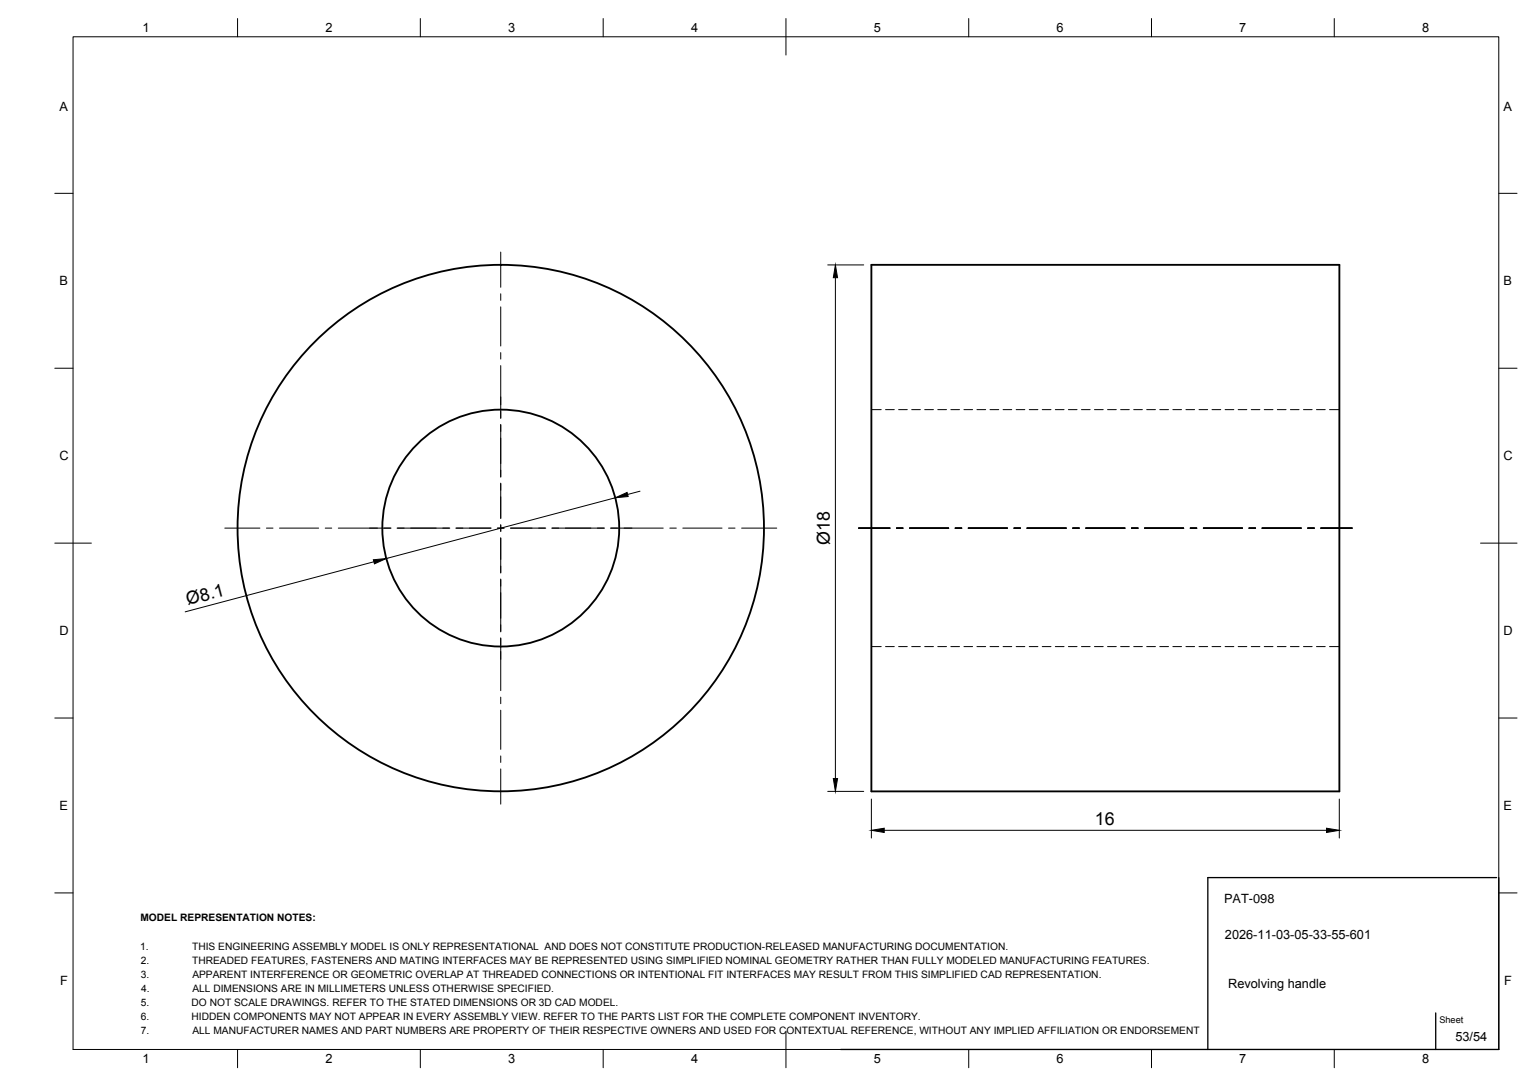
ISO-10303-21;
HEADER;
/* Generated by software containing ST-Developer
 * from STEP Tools, Inc. (www.steptools.com) 
 */

FILE_DESCRIPTION(
/* description */ ('Spring compression tester'),
/* implementation_level */ '2;1');

FILE_NAME(
/* name */ 'Revolving handle.step',
/* time_stamp */ '2026-10-28T03:24:11-07:00',
/* author */ (''),
/* organization */ (''),
/* preprocessor_version */ 'ST-DEVELOPER v20.2',
/* originating_system */ 'Autodesk Translation Framework v15.17.0.0',
/* authorisation */ '');

FILE_SCHEMA (('AUTOMOTIVE_DESIGN { 1 0 10303 214 3 1 1 }'));
ENDSEC;

DATA;
#10=MECHANICAL_DESIGN_GEOMETRIC_PRESENTATION_REPRESENTATION('',(#1174),#43521);
#1039=SHAPE_REPRESENTATION_RELATIONSHIP('SRR','None',#43856,#1099);
#1099=ADVANCED_BREP_SHAPE_REPRESENTATION('',(#1243),#43516);
#1174=STYLED_ITEM('',(#44195),#1243);
#1243=MANIFOLD_SOLID_BREP('Body1',#18617);
#1583=FACE_BOUND('',#4556,.T.);
#1584=FACE_BOUND('',#4558,.T.);
#2136=PLANE('',#21117);
#2137=PLANE('',#21118);
#3170=FACE_OUTER_BOUND('',#4553,.T.);
#3171=FACE_OUTER_BOUND('',#4554,.T.);
#3172=FACE_OUTER_BOUND('',#4555,.T.);
#3173=FACE_OUTER_BOUND('',#4557,.T.);
#4553=EDGE_LOOP('',(#16919,#16920,#16921,#16922));
#4554=EDGE_LOOP('',(#16923,#16924,#16925,#16926));
#4555=EDGE_LOOP('',(#16927));
#4556=EDGE_LOOP('',(#16928));
#4557=EDGE_LOOP('',(#16929));
#4558=EDGE_LOOP('',(#16930));
#5965=LINE('',#43172,#7397);
#5966=LINE('',#43178,#7398);
#7397=VECTOR('',#26213,0.405);
#7398=VECTOR('',#26220,0.9);
#8116=CIRCLE('',#21112,0.405);
#8117=CIRCLE('',#21113,0.405);
#8118=CIRCLE('',#21115,0.9);
#8119=CIRCLE('',#21116,0.9);
#9713=VERTEX_POINT('',#43169);
#9714=VERTEX_POINT('',#43171);
#9715=VERTEX_POINT('',#43175);
#9716=VERTEX_POINT('',#43177);
#12124=EDGE_CURVE('',#9713,#9713,#8116,.T.);
#12125=EDGE_CURVE('',#9713,#9714,#5965,.T.);
#12126=EDGE_CURVE('',#9714,#9714,#8117,.T.);
#12127=EDGE_CURVE('',#9715,#9715,#8118,.T.);
#12128=EDGE_CURVE('',#9715,#9716,#5966,.T.);
#12129=EDGE_CURVE('',#9716,#9716,#8119,.T.);
#16919=ORIENTED_EDGE('',*,*,#12124,.F.);
#16920=ORIENTED_EDGE('',*,*,#12125,.T.);
#16921=ORIENTED_EDGE('',*,*,#12126,.T.);
#16922=ORIENTED_EDGE('',*,*,#12125,.F.);
#16923=ORIENTED_EDGE('',*,*,#12127,.F.);
#16924=ORIENTED_EDGE('',*,*,#12128,.T.);
#16925=ORIENTED_EDGE('',*,*,#12129,.T.);
#16926=ORIENTED_EDGE('',*,*,#12128,.F.);
#16927=ORIENTED_EDGE('',*,*,#12127,.T.);
#16928=ORIENTED_EDGE('',*,*,#12124,.T.);
#16929=ORIENTED_EDGE('',*,*,#12129,.F.);
#16930=ORIENTED_EDGE('',*,*,#12126,.F.);
#17487=CYLINDRICAL_SURFACE('',#21111,0.405);
#17488=CYLINDRICAL_SURFACE('',#21114,0.9);
#18494=ADVANCED_FACE('',(#3170),#17487,.F.);
#18495=ADVANCED_FACE('',(#3171),#17488,.T.);
#18496=ADVANCED_FACE('',(#3172,#1583),#2136,.T.);
#18497=ADVANCED_FACE('',(#3173,#1584),#2137,.F.);
#18617=CLOSED_SHELL('',(#18494,#18495,#18496,#18497));
#21110=AXIS2_PLACEMENT_3D('',#43167,#26207,#26208);
#21111=AXIS2_PLACEMENT_3D('',#43168,#26209,#26210);
#21112=AXIS2_PLACEMENT_3D('',#43170,#26211,#26212);
#21113=AXIS2_PLACEMENT_3D('',#43173,#26214,#26215);
#21114=AXIS2_PLACEMENT_3D('',#43174,#26216,#26217);
#21115=AXIS2_PLACEMENT_3D('',#43176,#26218,#26219);
#21116=AXIS2_PLACEMENT_3D('',#43179,#26221,#26222);
#21117=AXIS2_PLACEMENT_3D('',#43180,#26223,#26224);
#21118=AXIS2_PLACEMENT_3D('',#43181,#26225,#26226);
#26207=DIRECTION('axis',(0.,0.,1.));
#26208=DIRECTION('refdir',(1.,0.,0.));
#26209=DIRECTION('center_axis',(1.,0.,0.));
#26210=DIRECTION('ref_axis',(0.,0.,-1.));
#26211=DIRECTION('center_axis',(-1.,0.,0.));
#26212=DIRECTION('ref_axis',(0.,0.,-1.));
#26213=DIRECTION('',(-1.,0.,0.));
#26214=DIRECTION('center_axis',(-1.,0.,0.));
#26215=DIRECTION('ref_axis',(0.,0.,-1.));
#26216=DIRECTION('center_axis',(1.,0.,0.));
#26217=DIRECTION('ref_axis',(0.,0.,-1.));
#26218=DIRECTION('center_axis',(1.,0.,0.));
#26219=DIRECTION('ref_axis',(0.,0.,-1.));
#26220=DIRECTION('',(-1.,0.,0.));
#26221=DIRECTION('center_axis',(1.,0.,0.));
#26222=DIRECTION('ref_axis',(0.,0.,-1.));
#26223=DIRECTION('center_axis',(1.,0.,0.));
#26224=DIRECTION('ref_axis',(0.,0.,-1.));
#26225=DIRECTION('center_axis',(1.,0.,0.));
#26226=DIRECTION('ref_axis',(0.,0.,-1.));
#43167=CARTESIAN_POINT('',(0.,0.,0.));
#43168=CARTESIAN_POINT('Origin',(29.4,0.,6.5));
#43169=CARTESIAN_POINT('',(31.,-4.95981953654678E-17,6.905));
#43170=CARTESIAN_POINT('Origin',(31.,0.,6.5));
#43171=CARTESIAN_POINT('',(29.4,-4.95981953654678E-17,6.905));
#43172=CARTESIAN_POINT('',(29.4,-4.95981953654678E-17,6.905));
#43173=CARTESIAN_POINT('Origin',(29.4,0.,6.5));
#43174=CARTESIAN_POINT('Origin',(29.4,0.,6.5));
#43175=CARTESIAN_POINT('',(31.,-1.10218211923262E-16,7.4));
#43176=CARTESIAN_POINT('Origin',(31.,0.,6.5));
#43177=CARTESIAN_POINT('',(29.4,-1.10218211923262E-16,7.4));
#43178=CARTESIAN_POINT('',(29.4,-1.10218211923262E-16,7.4));
#43179=CARTESIAN_POINT('Origin',(29.4,0.,6.5));
#43180=CARTESIAN_POINT('Origin',(31.,0.,6.5));
#43181=CARTESIAN_POINT('Origin',(29.4,0.,6.5));
#43448=UNCERTAINTY_MEASURE_WITH_UNIT(LENGTH_MEASURE(0.001),#43522,
'DISTANCE_ACCURACY_VALUE',
'Maximum model space distance between geometric entities at asserted c
onnectivities');
#43453=UNCERTAINTY_MEASURE_WITH_UNIT(LENGTH_MEASURE(0.001),#43522,
'DISTANCE_ACCURACY_VALUE',
'Maximum model space distance between geometric entities at asserted c
onnectivities');
#43516=(
GEOMETRIC_REPRESENTATION_CONTEXT(3)
GLOBAL_UNCERTAINTY_ASSIGNED_CONTEXT((#43448))
GLOBAL_UNIT_ASSIGNED_CONTEXT((#43522,#43524,#43525))
REPRESENTATION_CONTEXT('','3D')
);
#43521=(
GEOMETRIC_REPRESENTATION_CONTEXT(3)
GLOBAL_UNCERTAINTY_ASSIGNED_CONTEXT((#43453))
GLOBAL_UNIT_ASSIGNED_CONTEXT((#43522,#43524,#43525))
REPRESENTATION_CONTEXT('','3D')
);
#43522=(
LENGTH_UNIT()
NAMED_UNIT(*)
SI_UNIT(.CENTI.,.METRE.)
);
#43524=(
NAMED_UNIT(*)
PLANE_ANGLE_UNIT()
SI_UNIT($,.RADIAN.)
);
#43525=(
NAMED_UNIT(*)
SI_UNIT($,.STERADIAN.)
SOLID_ANGLE_UNIT()
);
#43588=SHAPE_DEFINITION_REPRESENTATION(#43775,#43856);
#43775=PRODUCT_DEFINITION_SHAPE('',$,#43924);
#43856=SHAPE_REPRESENTATION('',(#21110),#43516);
#43861=PRODUCT_DEFINITION_CONTEXT('part definition',#44064,'design');
#43924=PRODUCT_DEFINITION('Revolving handle','Revolving handle',#43991,
#43861);
#43991=PRODUCT_DEFINITION_FORMATION('',$,#44128);
#44064=APPLICATION_CONTEXT(
'Core Data for Automotive Mechanical Design Process');
#44065=PRODUCT_CONTEXT('part definition',#44064,'mechanical');
#44128=PRODUCT('Revolving handle','Revolving handle','Revolving handle',
(#44065));
#44189=COLOUR_RGB('Sky Blue',0.24,0.69,0.87);
#44190=FILL_AREA_STYLE_COLOUR('',#44189);
#44191=FILL_AREA_STYLE('',(#44190));
#44192=SURFACE_STYLE_FILL_AREA(#44191);
#44193=SURFACE_SIDE_STYLE('',(#44192));
#44194=SURFACE_STYLE_USAGE(.BOTH.,#44193);
#44195=PRESENTATION_STYLE_ASSIGNMENT((#44194));
ENDSEC;
END-ISO-10303-21;
